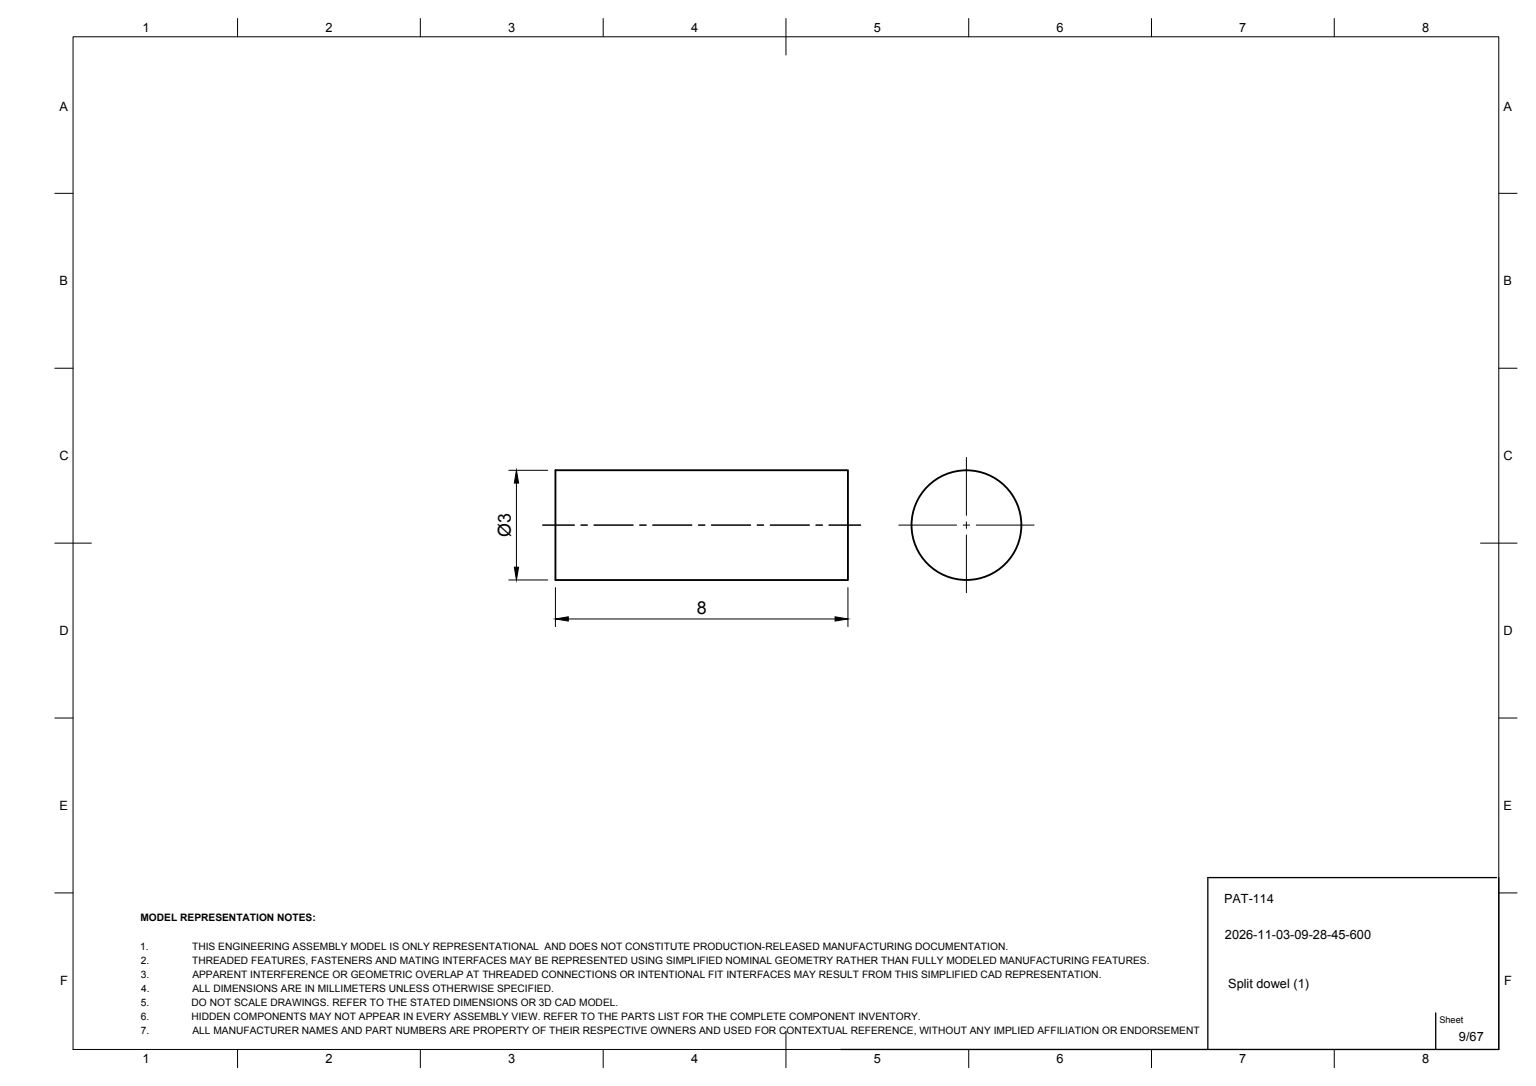
ISO-10303-21;
HEADER;
/* Generated by software containing ST-Developer
 * from STEP Tools, Inc. (www.steptools.com) 
 */

FILE_DESCRIPTION(
/* description */ ('Two-stage gear reducer in split housing'),
/* implementation_level */ '2;1');

FILE_NAME(
/* name */ 'Split dowel (1).step',
/* time_stamp */ '2026-10-28T03:22:31-07:00',
/* author */ (''),
/* organization */ (''),
/* preprocessor_version */ 'ST-DEVELOPER v20.2',
/* originating_system */ 'Autodesk Translation Framework v15.17.0.0',
/* authorisation */ '');

FILE_SCHEMA (('AUTOMOTIVE_DESIGN { 1 0 10303 214 3 1 1 }'));
ENDSEC;

DATA;
#10=MECHANICAL_DESIGN_GEOMETRIC_PRESENTATION_REPRESENTATION('',(#1238),#73366);
#1126=SHAPE_REPRESENTATION_RELATIONSHIP('SRR','None',#73613,#1182);
#1182=ADVANCED_BREP_SHAPE_REPRESENTATION('',(#1309),#73309);
#1238=STYLED_ITEM('',(#73974),#1309);
#1309=MANIFOLD_SOLID_BREP('Body1',#16126);
#1702=PLANE('',#17177);
#1703=PLANE('',#17178);
#2187=FACE_OUTER_BOUND('',#3186,.T.);
#2188=FACE_OUTER_BOUND('',#3187,.T.);
#2189=FACE_OUTER_BOUND('',#3188,.T.);
#3186=EDGE_LOOP('',(#11353,#11354,#11355,#11356));
#3187=EDGE_LOOP('',(#11357));
#3188=EDGE_LOOP('',(#11358));
#4309=LINE('',#23675,#5333);
#5333=VECTOR('',#19439,0.15);
#6274=CIRCLE('',#17175,0.15);
#6275=CIRCLE('',#17176,0.15);
#7106=VERTEX_POINT('',#23672);
#7107=VERTEX_POINT('',#23674);
#8730=EDGE_CURVE('',#7106,#7106,#6274,.T.);
#8731=EDGE_CURVE('',#7106,#7107,#4309,.T.);
#8732=EDGE_CURVE('',#7107,#7107,#6275,.T.);
#11353=ORIENTED_EDGE('',*,*,#8730,.F.);
#11354=ORIENTED_EDGE('',*,*,#8731,.T.);
#11355=ORIENTED_EDGE('',*,*,#8732,.T.);
#11356=ORIENTED_EDGE('',*,*,#8731,.F.);
#11357=ORIENTED_EDGE('',*,*,#8730,.T.);
#11358=ORIENTED_EDGE('',*,*,#8732,.F.);
#14992=CYLINDRICAL_SURFACE('',#17174,0.15);
#15394=ADVANCED_FACE('',(#2187),#14992,.T.);
#15395=ADVANCED_FACE('',(#2188),#1702,.T.);
#15396=ADVANCED_FACE('',(#2189),#1703,.F.);
#16126=CLOSED_SHELL('',(#15394,#15395,#15396));
#17173=AXIS2_PLACEMENT_3D('',#23670,#19433,#19434);
#17174=AXIS2_PLACEMENT_3D('',#23671,#19435,#19436);
#17175=AXIS2_PLACEMENT_3D('',#23673,#19437,#19438);
#17176=AXIS2_PLACEMENT_3D('',#23676,#19440,#19441);
#17177=AXIS2_PLACEMENT_3D('',#23677,#19442,#19443);
#17178=AXIS2_PLACEMENT_3D('',#23678,#19444,#19445);
#19433=DIRECTION('axis',(0.,0.,1.));
#19434=DIRECTION('refdir',(1.,0.,0.));
#19435=DIRECTION('center_axis',(0.,0.,1.));
#19436=DIRECTION('ref_axis',(1.,0.,0.));
#19437=DIRECTION('center_axis',(0.,0.,1.));
#19438=DIRECTION('ref_axis',(1.,0.,0.));
#19439=DIRECTION('',(0.,0.,-1.));
#19440=DIRECTION('center_axis',(0.,0.,1.));
#19441=DIRECTION('ref_axis',(1.,0.,0.));
#19442=DIRECTION('center_axis',(0.,0.,1.));
#19443=DIRECTION('ref_axis',(1.,0.,0.));
#19444=DIRECTION('center_axis',(0.,0.,1.));
#19445=DIRECTION('ref_axis',(1.,0.,0.));
#23670=CARTESIAN_POINT('',(0.,0.,0.));
#23671=CARTESIAN_POINT('Origin',(-4.75,3.,9.6));
#23672=CARTESIAN_POINT('',(-4.9,3.,10.4));
#23673=CARTESIAN_POINT('Origin',(-4.75,3.,10.4));
#23674=CARTESIAN_POINT('',(-4.9,3.,9.6));
#23675=CARTESIAN_POINT('',(-4.9,3.,9.6));
#23676=CARTESIAN_POINT('Origin',(-4.75,3.,9.6));
#23677=CARTESIAN_POINT('Origin',(-4.75,3.,10.4));
#23678=CARTESIAN_POINT('Origin',(-4.75,3.,9.6));
#73245=UNCERTAINTY_MEASURE_WITH_UNIT(LENGTH_MEASURE(0.001),#73367,
'DISTANCE_ACCURACY_VALUE',
'Maximum model space distance between geometric entities at asserted c
onnectivities');
#73302=UNCERTAINTY_MEASURE_WITH_UNIT(LENGTH_MEASURE(0.001),#73367,
'DISTANCE_ACCURACY_VALUE',
'Maximum model space distance between geometric entities at asserted c
onnectivities');
#73309=(
GEOMETRIC_REPRESENTATION_CONTEXT(3)
GLOBAL_UNCERTAINTY_ASSIGNED_CONTEXT((#73245))
GLOBAL_UNIT_ASSIGNED_CONTEXT((#73367,#73369,#73370))
REPRESENTATION_CONTEXT('','3D')
);
#73366=(
GEOMETRIC_REPRESENTATION_CONTEXT(3)
GLOBAL_UNCERTAINTY_ASSIGNED_CONTEXT((#73302))
GLOBAL_UNIT_ASSIGNED_CONTEXT((#73367,#73369,#73370))
REPRESENTATION_CONTEXT('','3D')
);
#73367=(
LENGTH_UNIT()
NAMED_UNIT(*)
SI_UNIT(.CENTI.,.METRE.)
);
#73369=(
NAMED_UNIT(*)
PLANE_ANGLE_UNIT()
SI_UNIT($,.RADIAN.)
);
#73370=(
NAMED_UNIT(*)
SI_UNIT($,.STERADIAN.)
SOLID_ANGLE_UNIT()
);
#73377=SHAPE_DEFINITION_REPRESENTATION(#73440,#73613);
#73440=PRODUCT_DEFINITION_SHAPE('',$,#73677);
#73613=SHAPE_REPRESENTATION('',(#17173),#73309);
#73670=PRODUCT_DEFINITION_CONTEXT('part definition',#73861,'design');
#73677=PRODUCT_DEFINITION('Split dowel (1)','Split dowel (1)',#73740,#73670);
#73740=PRODUCT_DEFINITION_FORMATION('',$,#73869);
#73861=APPLICATION_CONTEXT(
'Core Data for Automotive Mechanical Design Process');
#73862=PRODUCT_CONTEXT('part definition',#73861,'mechanical');
#73869=PRODUCT('Split dowel (1)','Split dowel (1)','Split dowel (1)',(#73862));
#73968=COLOUR_RGB('Light Blue',0.38,0.62,0.78);
#73969=FILL_AREA_STYLE_COLOUR('',#73968);
#73970=FILL_AREA_STYLE('',(#73969));
#73971=SURFACE_STYLE_FILL_AREA(#73970);
#73972=SURFACE_SIDE_STYLE('',(#73971));
#73973=SURFACE_STYLE_USAGE(.BOTH.,#73972);
#73974=PRESENTATION_STYLE_ASSIGNMENT((#73973));
ENDSEC;
END-ISO-10303-21;
